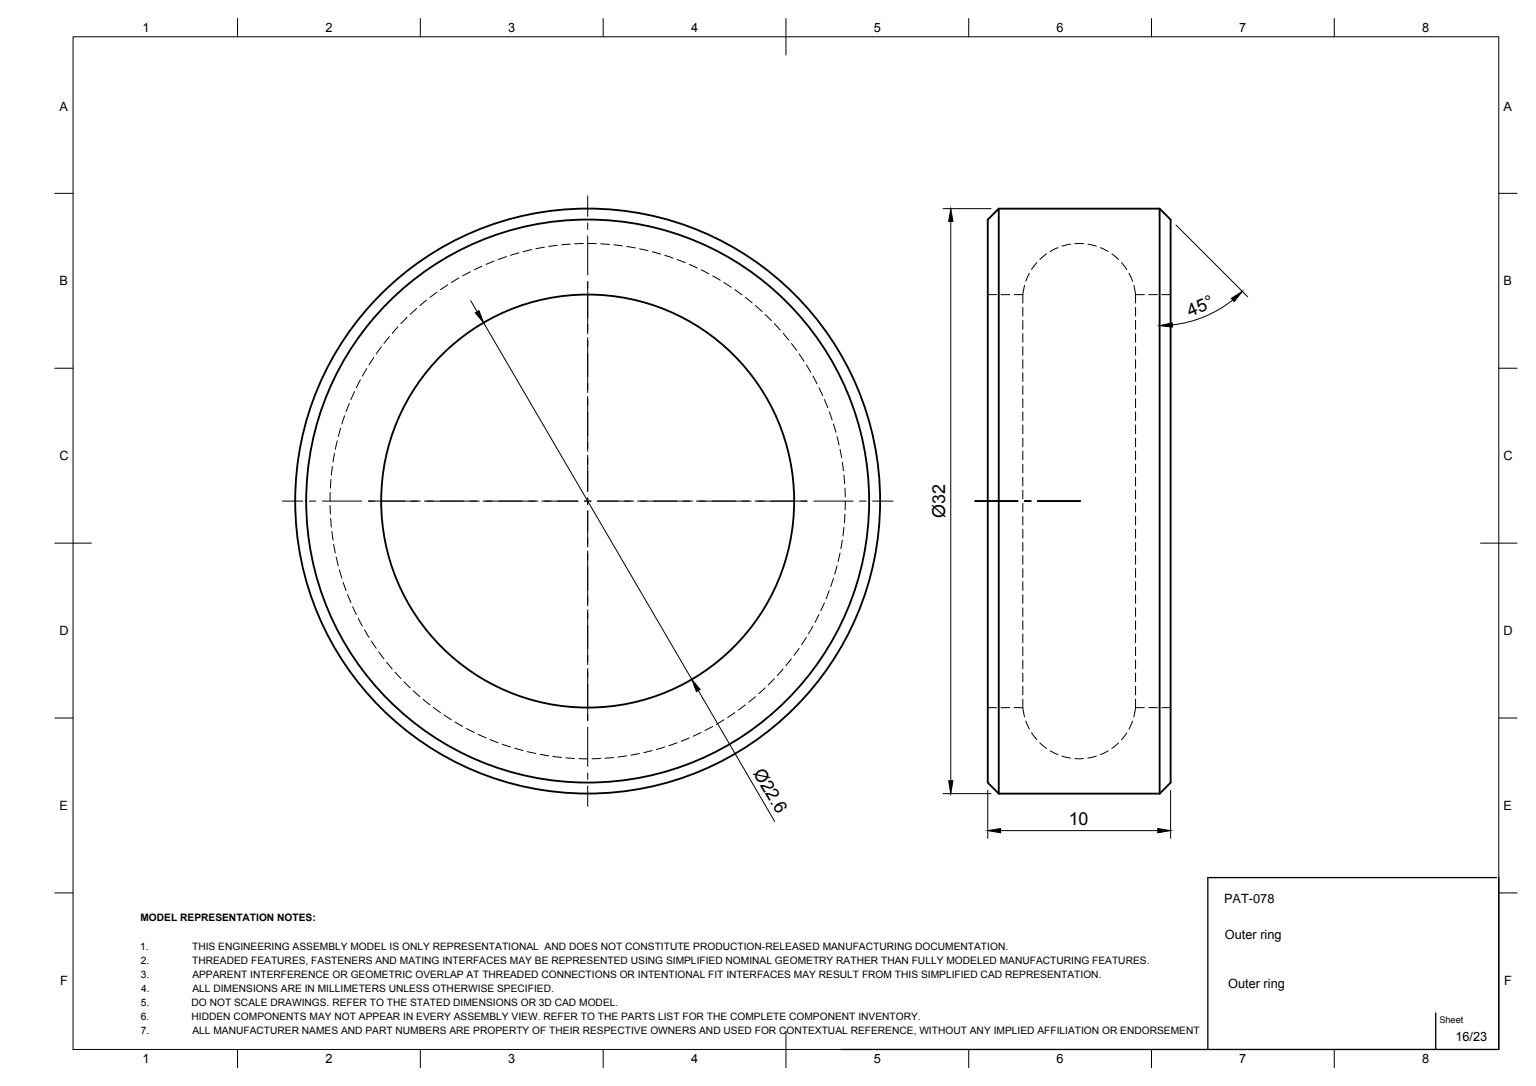
ISO-10303-21;
HEADER;
/* Generated by software containing ST-Developer
 * from STEP Tools, Inc. (www.steptools.com) 
 */

FILE_DESCRIPTION(
/* description */ ('Pedal-braked fixed caster'),
/* implementation_level */ '2;1');

FILE_NAME(
/* name */ 'Outer ring.step',
/* time_stamp */ '2026-10-28T03:26:52-07:00',
/* author */ (''),
/* organization */ (''),
/* preprocessor_version */ 'ST-DEVELOPER v20.2',
/* originating_system */ 'Autodesk Translation Framework v15.17.0.0',
/* authorisation */ '');

FILE_SCHEMA (('AUTOMOTIVE_DESIGN { 1 0 10303 214 3 1 1 }'));
ENDSEC;

DATA;
#10=MECHANICAL_DESIGN_GEOMETRIC_PRESENTATION_REPRESENTATION('',(#216),#5734);
#40=TOROIDAL_SURFACE('',#3409,1.1,0.309556);
#168=CONICAL_SURFACE('',#3420,1.57,0.785398163397449);
#169=CONICAL_SURFACE('',#3424,1.57,0.785398163397449);
#182=SHAPE_REPRESENTATION_RELATIONSHIP('SRR','None',#5822,#199);
#199=ADVANCED_BREP_SHAPE_REPRESENTATION('',(#239),#5726);
#216=STYLED_ITEM('',(#5984),#239);
#239=MANIFOLD_SOLID_BREP('Body1',#2998);
#281=CYLINDRICAL_SURFACE('',#3415,1.129765);
#282=CYLINDRICAL_SURFACE('',#3422,1.6);
#283=CYLINDRICAL_SURFACE('',#3427,1.129765);
#329=FACE_BOUND('',#807,.T.);
#330=FACE_BOUND('',#812,.T.);
#408=CIRCLE('',#3410,1.129765);
#409=CIRCLE('',#3411,1.129765);
#410=CIRCLE('',#3412,0.309556);
#411=CIRCLE('',#3413,1.129765);
#412=CIRCLE('',#3414,1.129765);
#413=CIRCLE('',#3416,1.129765);
#414=CIRCLE('',#3418,1.54);
#415=CIRCLE('',#3419,1.129765);
#416=CIRCLE('',#3421,1.6);
#417=CIRCLE('',#3423,1.6);
#418=CIRCLE('',#3425,1.54);
#592=FACE_OUTER_BOUND('',#804,.T.);
#593=FACE_OUTER_BOUND('',#805,.T.);
#594=FACE_OUTER_BOUND('',#806,.T.);
#595=FACE_OUTER_BOUND('',#808,.T.);
#596=FACE_OUTER_BOUND('',#809,.T.);
#597=FACE_OUTER_BOUND('',#810,.T.);
#598=FACE_OUTER_BOUND('',#811,.T.);
#599=FACE_OUTER_BOUND('',#813,.T.);
#804=EDGE_LOOP('',(#2438,#2439,#2440,#2441,#2442,#2443));
#805=EDGE_LOOP('',(#2444,#2445,#2446,#2447,#2448));
#806=EDGE_LOOP('',(#2449));
#807=EDGE_LOOP('',(#2450));
#808=EDGE_LOOP('',(#2451,#2452,#2453,#2454));
#809=EDGE_LOOP('',(#2455,#2456,#2457,#2458));
#810=EDGE_LOOP('',(#2459,#2460,#2461,#2462));
#811=EDGE_LOOP('',(#2463));
#812=EDGE_LOOP('',(#2464));
#813=EDGE_LOOP('',(#2465,#2466,#2467,#2468,#2469));
#1040=LINE('',#5097,#1252);
#1041=LINE('',#5106,#1253);
#1042=LINE('',#5110,#1254);
#1043=LINE('',#5114,#1255);
#1044=LINE('',#5117,#1256);
#1252=VECTOR('',#4158,1.129765);
#1253=VECTOR('',#4169,1.57);
#1254=VECTOR('',#4174,1.6);
#1255=VECTOR('',#4179,1.57);
#1256=VECTOR('',#4184,1.129765);
#1464=VERTEX_POINT('',#5085);
#1465=VERTEX_POINT('',#5086);
#1466=VERTEX_POINT('',#5089);
#1467=VERTEX_POINT('',#5091);
#1468=VERTEX_POINT('',#5095);
#1469=VERTEX_POINT('',#5099);
#1470=VERTEX_POINT('',#5101);
#1471=VERTEX_POINT('',#5104);
#1472=VERTEX_POINT('',#5108);
#1473=VERTEX_POINT('',#5112);
#1809=EDGE_CURVE('',#1464,#1465,#408,.T.);
#1810=EDGE_CURVE('',#1465,#1464,#409,.T.);
#1811=EDGE_CURVE('',#1465,#1466,#410,.T.);
#1812=EDGE_CURVE('',#1467,#1466,#411,.T.);
#1813=EDGE_CURVE('',#1466,#1467,#412,.T.);
#1814=EDGE_CURVE('',#1468,#1468,#413,.T.);
#1815=EDGE_CURVE('',#1468,#1467,#1040,.T.);
#1816=EDGE_CURVE('',#1469,#1469,#414,.T.);
#1817=EDGE_CURVE('',#1470,#1470,#415,.T.);
#1818=EDGE_CURVE('',#1471,#1471,#416,.T.);
#1819=EDGE_CURVE('',#1471,#1469,#1041,.T.);
#1820=EDGE_CURVE('',#1472,#1472,#417,.T.);
#1821=EDGE_CURVE('',#1472,#1471,#1042,.T.);
#1822=EDGE_CURVE('',#1473,#1473,#418,.T.);
#1823=EDGE_CURVE('',#1473,#1472,#1043,.T.);
#1824=EDGE_CURVE('',#1464,#1470,#1044,.T.);
#2438=ORIENTED_EDGE('',*,*,#1809,.F.);
#2439=ORIENTED_EDGE('',*,*,#1810,.F.);
#2440=ORIENTED_EDGE('',*,*,#1811,.T.);
#2441=ORIENTED_EDGE('',*,*,#1812,.F.);
#2442=ORIENTED_EDGE('',*,*,#1813,.F.);
#2443=ORIENTED_EDGE('',*,*,#1811,.F.);
#2444=ORIENTED_EDGE('',*,*,#1814,.T.);
#2445=ORIENTED_EDGE('',*,*,#1815,.T.);
#2446=ORIENTED_EDGE('',*,*,#1812,.T.);
#2447=ORIENTED_EDGE('',*,*,#1813,.T.);
#2448=ORIENTED_EDGE('',*,*,#1815,.F.);
#2449=ORIENTED_EDGE('',*,*,#1816,.F.);
#2450=ORIENTED_EDGE('',*,*,#1817,.T.);
#2451=ORIENTED_EDGE('',*,*,#1818,.F.);
#2452=ORIENTED_EDGE('',*,*,#1819,.T.);
#2453=ORIENTED_EDGE('',*,*,#1816,.T.);
#2454=ORIENTED_EDGE('',*,*,#1819,.F.);
#2455=ORIENTED_EDGE('',*,*,#1820,.F.);
#2456=ORIENTED_EDGE('',*,*,#1821,.T.);
#2457=ORIENTED_EDGE('',*,*,#1818,.T.);
#2458=ORIENTED_EDGE('',*,*,#1821,.F.);
#2459=ORIENTED_EDGE('',*,*,#1822,.F.);
#2460=ORIENTED_EDGE('',*,*,#1823,.T.);
#2461=ORIENTED_EDGE('',*,*,#1820,.T.);
#2462=ORIENTED_EDGE('',*,*,#1823,.F.);
#2463=ORIENTED_EDGE('',*,*,#1822,.T.);
#2464=ORIENTED_EDGE('',*,*,#1814,.F.);
#2465=ORIENTED_EDGE('',*,*,#1809,.T.);
#2466=ORIENTED_EDGE('',*,*,#1810,.T.);
#2467=ORIENTED_EDGE('',*,*,#1824,.T.);
#2468=ORIENTED_EDGE('',*,*,#1817,.F.);
#2469=ORIENTED_EDGE('',*,*,#1824,.F.);
#2778=PLANE('',#3417);
#2779=PLANE('',#3426);
#2925=ADVANCED_FACE('',(#592),#40,.F.);
#2926=ADVANCED_FACE('',(#593),#281,.F.);
#2927=ADVANCED_FACE('',(#594,#329),#2778,.T.);
#2928=ADVANCED_FACE('',(#595),#168,.T.);
#2929=ADVANCED_FACE('',(#596),#282,.T.);
#2930=ADVANCED_FACE('',(#597),#169,.T.);
#2931=ADVANCED_FACE('',(#598,#330),#2779,.T.);
#2932=ADVANCED_FACE('',(#599),#283,.F.);
#2998=CLOSED_SHELL('',(#2925,#2926,#2927,#2928,#2929,#2930,#2931,#2932));
#3408=AXIS2_PLACEMENT_3D('',#5083,#4140,#4141);
#3409=AXIS2_PLACEMENT_3D('',#5084,#4142,#4143);
#3410=AXIS2_PLACEMENT_3D('',#5087,#4144,#4145);
#3411=AXIS2_PLACEMENT_3D('',#5088,#4146,#4147);
#3412=AXIS2_PLACEMENT_3D('',#5090,#4148,#4149);
#3413=AXIS2_PLACEMENT_3D('',#5092,#4150,#4151);
#3414=AXIS2_PLACEMENT_3D('',#5093,#4152,#4153);
#3415=AXIS2_PLACEMENT_3D('',#5094,#4154,#4155);
#3416=AXIS2_PLACEMENT_3D('',#5096,#4156,#4157);
#3417=AXIS2_PLACEMENT_3D('',#5098,#4159,#4160);
#3418=AXIS2_PLACEMENT_3D('',#5100,#4161,#4162);
#3419=AXIS2_PLACEMENT_3D('',#5102,#4163,#4164);
#3420=AXIS2_PLACEMENT_3D('',#5103,#4165,#4166);
#3421=AXIS2_PLACEMENT_3D('',#5105,#4167,#4168);
#3422=AXIS2_PLACEMENT_3D('',#5107,#4170,#4171);
#3423=AXIS2_PLACEMENT_3D('',#5109,#4172,#4173);
#3424=AXIS2_PLACEMENT_3D('',#5111,#4175,#4176);
#3425=AXIS2_PLACEMENT_3D('',#5113,#4177,#4178);
#3426=AXIS2_PLACEMENT_3D('',#5115,#4180,#4181);
#3427=AXIS2_PLACEMENT_3D('',#5116,#4182,#4183);
#4140=DIRECTION('axis',(0.,0.,1.));
#4141=DIRECTION('refdir',(1.,0.,0.));
#4142=DIRECTION('center_axis',(0.,-1.,0.));
#4143=DIRECTION('ref_axis',(0.,0.,-1.));
#4144=DIRECTION('center_axis',(0.,-1.,0.));
#4145=DIRECTION('ref_axis',(1.,0.,0.));
#4146=DIRECTION('center_axis',(0.,-1.,0.));
#4147=DIRECTION('ref_axis',(1.,0.,0.));
#4148=DIRECTION('center_axis',(1.,0.,1.22464679914735E-16));
#4149=DIRECTION('ref_axis',(-1.22464679914735E-16,0.,1.));
#4150=DIRECTION('center_axis',(0.,1.,0.));
#4151=DIRECTION('ref_axis',(1.,0.,0.));
#4152=DIRECTION('center_axis',(0.,1.,0.));
#4153=DIRECTION('ref_axis',(1.,0.,0.));
#4154=DIRECTION('center_axis',(0.,-1.,0.));
#4155=DIRECTION('ref_axis',(1.,0.,0.));
#4156=DIRECTION('center_axis',(0.,-1.,0.));
#4157=DIRECTION('ref_axis',(1.,0.,0.));
#4158=DIRECTION('',(0.,1.,0.));
#4159=DIRECTION('center_axis',(0.,1.,0.));
#4160=DIRECTION('ref_axis',(0.,0.,1.));
#4161=DIRECTION('center_axis',(0.,-1.,0.));
#4162=DIRECTION('ref_axis',(1.,0.,0.));
#4163=DIRECTION('center_axis',(0.,-1.,0.));
#4164=DIRECTION('ref_axis',(1.,0.,0.));
#4165=DIRECTION('center_axis',(0.,-1.,0.));
#4166=DIRECTION('ref_axis',(1.,0.,0.));
#4167=DIRECTION('center_axis',(0.,-1.,0.));
#4168=DIRECTION('ref_axis',(1.,0.,0.));
#4169=DIRECTION('',(0.707106781186548,0.707106781186547,8.65956056235494E-17));
#4170=DIRECTION('center_axis',(0.,-1.,0.));
#4171=DIRECTION('ref_axis',(1.,0.,0.));
#4172=DIRECTION('center_axis',(0.,-1.,0.));
#4173=DIRECTION('ref_axis',(1.,0.,0.));
#4174=DIRECTION('',(0.,1.,0.));
#4175=DIRECTION('center_axis',(0.,1.,0.));
#4176=DIRECTION('ref_axis',(1.,0.,0.));
#4177=DIRECTION('center_axis',(0.,-1.,0.));
#4178=DIRECTION('ref_axis',(1.,0.,0.));
#4179=DIRECTION('',(-0.707106781186548,0.707106781186547,-8.65956056235494E-17));
#4180=DIRECTION('center_axis',(0.,-1.,0.));
#4181=DIRECTION('ref_axis',(0.,0.,-1.));
#4182=DIRECTION('center_axis',(0.,-1.,0.));
#4183=DIRECTION('ref_axis',(1.,0.,0.));
#4184=DIRECTION('',(0.,1.,0.));
#5083=CARTESIAN_POINT('',(0.,0.,0.));
#5084=CARTESIAN_POINT('Origin',(0.,0.,0.));
#5085=CARTESIAN_POINT('',(-1.129765,0.308121667383195,-1.38356309103871E-16));
#5086=CARTESIAN_POINT('',(-1.38356309103871E-16,0.308121667383195,1.129765));
#5087=CARTESIAN_POINT('Origin',(0.,0.308121667383195,0.));
#5088=CARTESIAN_POINT('Origin',(0.,0.308121667383195,0.));
#5089=CARTESIAN_POINT('',(-1.38356309103871E-16,-0.308121667383195,1.129765));
#5090=CARTESIAN_POINT('Origin',(-1.34711147906209E-16,0.,1.1));
#5091=CARTESIAN_POINT('',(-1.129765,-0.308121667383195,1.38356309103871E-16));
#5092=CARTESIAN_POINT('Origin',(0.,-0.308121667383195,0.));
#5093=CARTESIAN_POINT('Origin',(0.,-0.308121667383195,0.));
#5094=CARTESIAN_POINT('Origin',(0.,0.,0.));
#5095=CARTESIAN_POINT('',(-1.129765,-0.5,-1.38356309103871E-16));
#5096=CARTESIAN_POINT('Origin',(0.,-0.5,0.));
#5097=CARTESIAN_POINT('',(-1.129765,0.,-1.38356309103871E-16));
#5098=CARTESIAN_POINT('Origin',(1.54,0.5,0.));
#5099=CARTESIAN_POINT('',(-1.54,0.5,-1.88595607068692E-16));
#5100=CARTESIAN_POINT('Origin',(0.,0.5,0.));
#5101=CARTESIAN_POINT('',(-1.129765,0.5,-1.38356309103871E-16));
#5102=CARTESIAN_POINT('Origin',(0.,0.5,0.));
#5103=CARTESIAN_POINT('Origin',(0.,0.47,0.));
#5104=CARTESIAN_POINT('',(-1.6,0.44,-1.95943487863577E-16));
#5105=CARTESIAN_POINT('Origin',(0.,0.44,0.));
#5106=CARTESIAN_POINT('',(-1.57,0.47,-1.92269547466134E-16));
#5107=CARTESIAN_POINT('Origin',(0.,0.,0.));
#5108=CARTESIAN_POINT('',(-1.6,-0.44,-1.95943487863577E-16));
#5109=CARTESIAN_POINT('Origin',(0.,-0.44,0.));
#5110=CARTESIAN_POINT('',(-1.6,0.,-1.95943487863577E-16));
#5111=CARTESIAN_POINT('Origin',(0.,-0.47,0.));
#5112=CARTESIAN_POINT('',(-1.54,-0.5,-1.88595607068692E-16));
#5113=CARTESIAN_POINT('Origin',(0.,-0.5,0.));
#5114=CARTESIAN_POINT('',(-1.57,-0.47,-1.92269547466134E-16));
#5115=CARTESIAN_POINT('Origin',(1.129765,-0.5,0.));
#5116=CARTESIAN_POINT('Origin',(0.,0.,0.));
#5117=CARTESIAN_POINT('',(-1.129765,0.,-1.38356309103871E-16));
#5703=UNCERTAINTY_MEASURE_WITH_UNIT(LENGTH_MEASURE(0.001),#5735,
'DISTANCE_ACCURACY_VALUE',
'Maximum model space distance between geometric entities at asserted c
onnectivities');
#5711=UNCERTAINTY_MEASURE_WITH_UNIT(LENGTH_MEASURE(0.001),#5735,
'DISTANCE_ACCURACY_VALUE',
'Maximum model space distance between geometric entities at asserted c
onnectivities');
#5726=(
GEOMETRIC_REPRESENTATION_CONTEXT(3)
GLOBAL_UNCERTAINTY_ASSIGNED_CONTEXT((#5703))
GLOBAL_UNIT_ASSIGNED_CONTEXT((#5735,#5737,#5738))
REPRESENTATION_CONTEXT('','3D')
);
#5734=(
GEOMETRIC_REPRESENTATION_CONTEXT(3)
GLOBAL_UNCERTAINTY_ASSIGNED_CONTEXT((#5711))
GLOBAL_UNIT_ASSIGNED_CONTEXT((#5735,#5737,#5738))
REPRESENTATION_CONTEXT('','3D')
);
#5735=(
LENGTH_UNIT()
NAMED_UNIT(*)
SI_UNIT(.CENTI.,.METRE.)
);
#5737=(
NAMED_UNIT(*)
PLANE_ANGLE_UNIT()
SI_UNIT($,.RADIAN.)
);
#5738=(
NAMED_UNIT(*)
SI_UNIT($,.STERADIAN.)
SOLID_ANGLE_UNIT()
);
#5753=SHAPE_DEFINITION_REPRESENTATION(#5785,#5822);
#5785=PRODUCT_DEFINITION_SHAPE('',$,#5845);
#5822=SHAPE_REPRESENTATION('',(#3408),#5726);
#5830=PRODUCT_DEFINITION_CONTEXT('part definition',#5898,'design');
#5845=PRODUCT_DEFINITION('Outer ring','Outer ring',#5867,#5830);
#5867=PRODUCT_DEFINITION_FORMATION('',$,#5914);
#5898=APPLICATION_CONTEXT(
'Core Data for Automotive Mechanical Design Process');
#5899=PRODUCT_CONTEXT('part definition',#5898,'mechanical');
#5914=PRODUCT('Outer ring','Outer ring','Outer ring',(#5899));
#5978=COLOUR_RGB('Grey',0.48,0.52,0.57);
#5979=FILL_AREA_STYLE_COLOUR('',#5978);
#5980=FILL_AREA_STYLE('',(#5979));
#5981=SURFACE_STYLE_FILL_AREA(#5980);
#5982=SURFACE_SIDE_STYLE('',(#5981));
#5983=SURFACE_STYLE_USAGE(.BOTH.,#5982);
#5984=PRESENTATION_STYLE_ASSIGNMENT((#5983));
ENDSEC;
END-ISO-10303-21;
